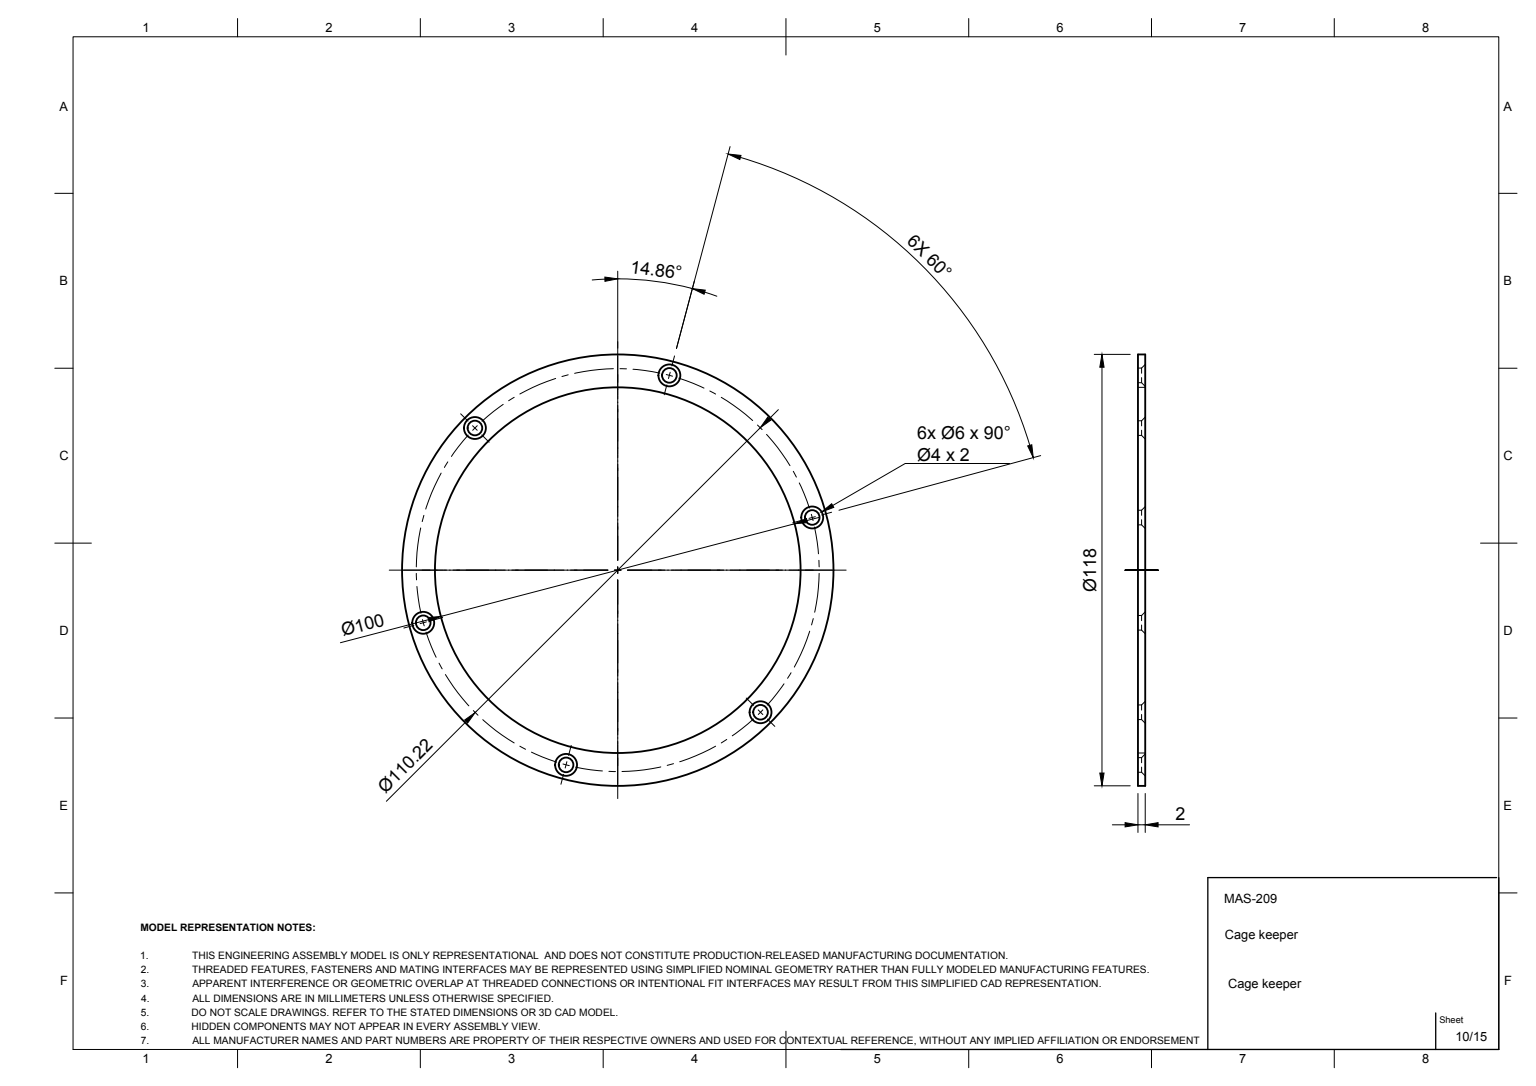
ISO-10303-21;
HEADER;
/* Generated by software containing ST-Developer
 * from STEP Tools, Inc. (www.steptools.com) 
 */

FILE_DESCRIPTION(
/* description */ ('Independent bearing-supported roller-ramp one-way clutch. Six logarit
hmic ramps with plain solid rollers, sprung guided plungers, native Co
il variants, removable shared keepers, rounded parallel key, shaft wit
h complete retaining lips, bronze journal/thrust support and bolted co
vers. Native rotor, roller planar/spin and plunger joints permit manua
l geometric engaged/released inspection. Automatic frictional torque s
witching/contact dynamics are not simulated; no capacity, hardness, fi
t, lubrication, speed, force or life rating. External input driver/cou
pling/anchors outside assembly.'),
/* implementation_level */ '2;1');

FILE_NAME(
/* name */ 'Cage keeper.step',
/* time_stamp */ '2026-11-08T07:04:38-08:00',
/* author */ (''),
/* organization */ (''),
/* preprocessor_version */ 'ST-DEVELOPER v20.2',
/* originating_system */ 'Autodesk Translation Framework v15.17.0.0',
/* authorisation */ '');

FILE_SCHEMA (('AUTOMOTIVE_DESIGN { 1 0 10303 214 3 1 1 }'));
ENDSEC;

DATA;
#10=MECHANICAL_DESIGN_GEOMETRIC_PRESENTATION_REPRESENTATION('',(#307),#99526);
#247=CONICAL_SURFACE('',#19556,2.5,0.785398163397448);
#248=CONICAL_SURFACE('',#19561,2.5,0.785398163397448);
#249=CONICAL_SURFACE('',#19566,2.5,0.785398163397448);
#250=CONICAL_SURFACE('',#19571,2.5,0.785398163397448);
#251=CONICAL_SURFACE('',#19576,2.5,0.785398163397448);
#252=CONICAL_SURFACE('',#19581,2.5,0.785398163397448);
#275=SHAPE_REPRESENTATION_RELATIONSHIP('SRR','None',#99632,#291);
#291=ADVANCED_BREP_SHAPE_REPRESENTATION('',(#323),#99517);
#307=STYLED_ITEM('',(#99715),#323);
#323=MANIFOLD_SOLID_BREP('Body1',#18277);
#416=FACE_BOUND('',#2646,.T.);
#417=FACE_BOUND('',#2647,.T.);
#418=FACE_BOUND('',#2648,.T.);
#419=FACE_BOUND('',#2649,.T.);
#420=FACE_BOUND('',#2650,.T.);
#421=FACE_BOUND('',#2651,.T.);
#422=FACE_BOUND('',#2652,.T.);
#423=FACE_BOUND('',#2654,.T.);
#424=FACE_BOUND('',#2655,.T.);
#425=FACE_BOUND('',#2656,.T.);
#426=FACE_BOUND('',#2657,.T.);
#427=FACE_BOUND('',#2658,.T.);
#428=FACE_BOUND('',#2659,.T.);
#429=FACE_BOUND('',#2660,.T.);
#577=PLANE('',#19592);
#578=PLANE('',#19593);
#1550=FACE_OUTER_BOUND('',#2631,.T.);
#1551=FACE_OUTER_BOUND('',#2632,.T.);
#1552=FACE_OUTER_BOUND('',#2633,.T.);
#1553=FACE_OUTER_BOUND('',#2634,.T.);
#1554=FACE_OUTER_BOUND('',#2635,.T.);
#1555=FACE_OUTER_BOUND('',#2636,.T.);
#1556=FACE_OUTER_BOUND('',#2637,.T.);
#1557=FACE_OUTER_BOUND('',#2638,.T.);
#1558=FACE_OUTER_BOUND('',#2639,.T.);
#1559=FACE_OUTER_BOUND('',#2640,.T.);
#1560=FACE_OUTER_BOUND('',#2641,.T.);
#1561=FACE_OUTER_BOUND('',#2642,.T.);
#1562=FACE_OUTER_BOUND('',#2643,.T.);
#1563=FACE_OUTER_BOUND('',#2644,.T.);
#1564=FACE_OUTER_BOUND('',#2645,.T.);
#1565=FACE_OUTER_BOUND('',#2653,.T.);
#2631=EDGE_LOOP('',(#15948,#15949,#15950,#15951));
#2632=EDGE_LOOP('',(#15952,#15953,#15954,#15955));
#2633=EDGE_LOOP('',(#15956,#15957,#15958,#15959));
#2634=EDGE_LOOP('',(#15960,#15961,#15962,#15963));
#2635=EDGE_LOOP('',(#15964,#15965,#15966,#15967));
#2636=EDGE_LOOP('',(#15968,#15969,#15970,#15971));
#2637=EDGE_LOOP('',(#15972,#15973,#15974,#15975));
#2638=EDGE_LOOP('',(#15976,#15977,#15978,#15979));
#2639=EDGE_LOOP('',(#15980,#15981,#15982,#15983));
#2640=EDGE_LOOP('',(#15984,#15985,#15986,#15987));
#2641=EDGE_LOOP('',(#15988,#15989,#15990,#15991));
#2642=EDGE_LOOP('',(#15992,#15993,#15994,#15995));
#2643=EDGE_LOOP('',(#15996,#15997,#15998,#15999));
#2644=EDGE_LOOP('',(#16000,#16001,#16002,#16003));
#2645=EDGE_LOOP('',(#16004));
#2646=EDGE_LOOP('',(#16005));
#2647=EDGE_LOOP('',(#16006));
#2648=EDGE_LOOP('',(#16007));
#2649=EDGE_LOOP('',(#16008));
#2650=EDGE_LOOP('',(#16009));
#2651=EDGE_LOOP('',(#16010));
#2652=EDGE_LOOP('',(#16011));
#2653=EDGE_LOOP('',(#16012));
#2654=EDGE_LOOP('',(#16013));
#2655=EDGE_LOOP('',(#16014));
#2656=EDGE_LOOP('',(#16015));
#2657=EDGE_LOOP('',(#16016));
#2658=EDGE_LOOP('',(#16017));
#2659=EDGE_LOOP('',(#16018));
#2660=EDGE_LOOP('',(#16019));
#3054=CIRCLE('',#19557,3.);
#3055=CIRCLE('',#19558,2.);
#3056=CIRCLE('',#19560,2.);
#3057=CIRCLE('',#19562,3.);
#3058=CIRCLE('',#19563,2.);
#3059=CIRCLE('',#19565,2.);
#3060=CIRCLE('',#19567,3.);
#3061=CIRCLE('',#19568,2.);
#3062=CIRCLE('',#19570,2.);
#3063=CIRCLE('',#19572,3.);
#3064=CIRCLE('',#19573,2.);
#3065=CIRCLE('',#19575,2.);
#3066=CIRCLE('',#19577,3.);
#3067=CIRCLE('',#19578,2.);
#3068=CIRCLE('',#19580,2.);
#3069=CIRCLE('',#19582,3.);
#3070=CIRCLE('',#19583,2.);
#3071=CIRCLE('',#19585,2.);
#3072=CIRCLE('',#19587,50.);
#3073=CIRCLE('',#19588,50.);
#3074=CIRCLE('',#19590,59.);
#3075=CIRCLE('',#19591,59.);
#5416=LINE('',#94779,#6320);
#5417=LINE('',#94783,#6321);
#5418=LINE('',#94789,#6322);
#5419=LINE('',#94793,#6323);
#5420=LINE('',#94799,#6324);
#5421=LINE('',#94803,#6325);
#5422=LINE('',#94809,#6326);
#5423=LINE('',#94813,#6327);
#5424=LINE('',#94819,#6328);
#5425=LINE('',#94823,#6329);
#5426=LINE('',#94829,#6330);
#5427=LINE('',#94833,#6331);
#5428=LINE('',#94839,#6332);
#5429=LINE('',#94845,#6333);
#6320=VECTOR('',#22775,2.5);
#6321=VECTOR('',#22780,2.);
#6322=VECTOR('',#22787,2.5);
#6323=VECTOR('',#22792,2.);
#6324=VECTOR('',#22799,2.5);
#6325=VECTOR('',#22804,2.);
#6326=VECTOR('',#22811,2.5);
#6327=VECTOR('',#22816,2.);
#6328=VECTOR('',#22823,2.5);
#6329=VECTOR('',#22828,2.);
#6330=VECTOR('',#22835,2.5);
#6331=VECTOR('',#22840,2.);
#6332=VECTOR('',#22847,50.);
#6333=VECTOR('',#22854,59.);
#8069=VERTEX_POINT('',#94776);
#8070=VERTEX_POINT('',#94778);
#8071=VERTEX_POINT('',#94782);
#8072=VERTEX_POINT('',#94786);
#8073=VERTEX_POINT('',#94788);
#8074=VERTEX_POINT('',#94792);
#8075=VERTEX_POINT('',#94796);
#8076=VERTEX_POINT('',#94798);
#8077=VERTEX_POINT('',#94802);
#8078=VERTEX_POINT('',#94806);
#8079=VERTEX_POINT('',#94808);
#8080=VERTEX_POINT('',#94812);
#8081=VERTEX_POINT('',#94816);
#8082=VERTEX_POINT('',#94818);
#8083=VERTEX_POINT('',#94822);
#8084=VERTEX_POINT('',#94826);
#8085=VERTEX_POINT('',#94828);
#8086=VERTEX_POINT('',#94832);
#8087=VERTEX_POINT('',#94836);
#8088=VERTEX_POINT('',#94838);
#8089=VERTEX_POINT('',#94842);
#8090=VERTEX_POINT('',#94844);
#10726=EDGE_CURVE('',#8069,#8069,#3054,.T.);
#10727=EDGE_CURVE('',#8069,#8070,#5416,.T.);
#10728=EDGE_CURVE('',#8070,#8070,#3055,.T.);
#10729=EDGE_CURVE('',#8070,#8071,#5417,.T.);
#10730=EDGE_CURVE('',#8071,#8071,#3056,.T.);
#10731=EDGE_CURVE('',#8072,#8072,#3057,.T.);
#10732=EDGE_CURVE('',#8072,#8073,#5418,.T.);
#10733=EDGE_CURVE('',#8073,#8073,#3058,.T.);
#10734=EDGE_CURVE('',#8073,#8074,#5419,.T.);
#10735=EDGE_CURVE('',#8074,#8074,#3059,.T.);
#10736=EDGE_CURVE('',#8075,#8075,#3060,.T.);
#10737=EDGE_CURVE('',#8075,#8076,#5420,.T.);
#10738=EDGE_CURVE('',#8076,#8076,#3061,.T.);
#10739=EDGE_CURVE('',#8076,#8077,#5421,.T.);
#10740=EDGE_CURVE('',#8077,#8077,#3062,.T.);
#10741=EDGE_CURVE('',#8078,#8078,#3063,.T.);
#10742=EDGE_CURVE('',#8078,#8079,#5422,.T.);
#10743=EDGE_CURVE('',#8079,#8079,#3064,.T.);
#10744=EDGE_CURVE('',#8079,#8080,#5423,.T.);
#10745=EDGE_CURVE('',#8080,#8080,#3065,.T.);
#10746=EDGE_CURVE('',#8081,#8081,#3066,.T.);
#10747=EDGE_CURVE('',#8081,#8082,#5424,.T.);
#10748=EDGE_CURVE('',#8082,#8082,#3067,.T.);
#10749=EDGE_CURVE('',#8082,#8083,#5425,.T.);
#10750=EDGE_CURVE('',#8083,#8083,#3068,.T.);
#10751=EDGE_CURVE('',#8084,#8084,#3069,.T.);
#10752=EDGE_CURVE('',#8084,#8085,#5426,.T.);
#10753=EDGE_CURVE('',#8085,#8085,#3070,.T.);
#10754=EDGE_CURVE('',#8085,#8086,#5427,.T.);
#10755=EDGE_CURVE('',#8086,#8086,#3071,.T.);
#10756=EDGE_CURVE('',#8087,#8087,#3072,.T.);
#10757=EDGE_CURVE('',#8087,#8088,#5428,.T.);
#10758=EDGE_CURVE('',#8088,#8088,#3073,.T.);
#10759=EDGE_CURVE('',#8089,#8089,#3074,.T.);
#10760=EDGE_CURVE('',#8089,#8090,#5429,.T.);
#10761=EDGE_CURVE('',#8090,#8090,#3075,.T.);
#15948=ORIENTED_EDGE('',*,*,#10726,.F.);
#15949=ORIENTED_EDGE('',*,*,#10727,.T.);
#15950=ORIENTED_EDGE('',*,*,#10728,.T.);
#15951=ORIENTED_EDGE('',*,*,#10727,.F.);
#15952=ORIENTED_EDGE('',*,*,#10728,.F.);
#15953=ORIENTED_EDGE('',*,*,#10729,.T.);
#15954=ORIENTED_EDGE('',*,*,#10730,.F.);
#15955=ORIENTED_EDGE('',*,*,#10729,.F.);
#15956=ORIENTED_EDGE('',*,*,#10731,.F.);
#15957=ORIENTED_EDGE('',*,*,#10732,.T.);
#15958=ORIENTED_EDGE('',*,*,#10733,.T.);
#15959=ORIENTED_EDGE('',*,*,#10732,.F.);
#15960=ORIENTED_EDGE('',*,*,#10733,.F.);
#15961=ORIENTED_EDGE('',*,*,#10734,.T.);
#15962=ORIENTED_EDGE('',*,*,#10735,.F.);
#15963=ORIENTED_EDGE('',*,*,#10734,.F.);
#15964=ORIENTED_EDGE('',*,*,#10736,.F.);
#15965=ORIENTED_EDGE('',*,*,#10737,.T.);
#15966=ORIENTED_EDGE('',*,*,#10738,.T.);
#15967=ORIENTED_EDGE('',*,*,#10737,.F.);
#15968=ORIENTED_EDGE('',*,*,#10738,.F.);
#15969=ORIENTED_EDGE('',*,*,#10739,.T.);
#15970=ORIENTED_EDGE('',*,*,#10740,.F.);
#15971=ORIENTED_EDGE('',*,*,#10739,.F.);
#15972=ORIENTED_EDGE('',*,*,#10741,.F.);
#15973=ORIENTED_EDGE('',*,*,#10742,.T.);
#15974=ORIENTED_EDGE('',*,*,#10743,.T.);
#15975=ORIENTED_EDGE('',*,*,#10742,.F.);
#15976=ORIENTED_EDGE('',*,*,#10743,.F.);
#15977=ORIENTED_EDGE('',*,*,#10744,.T.);
#15978=ORIENTED_EDGE('',*,*,#10745,.F.);
#15979=ORIENTED_EDGE('',*,*,#10744,.F.);
#15980=ORIENTED_EDGE('',*,*,#10746,.F.);
#15981=ORIENTED_EDGE('',*,*,#10747,.T.);
#15982=ORIENTED_EDGE('',*,*,#10748,.T.);
#15983=ORIENTED_EDGE('',*,*,#10747,.F.);
#15984=ORIENTED_EDGE('',*,*,#10748,.F.);
#15985=ORIENTED_EDGE('',*,*,#10749,.T.);
#15986=ORIENTED_EDGE('',*,*,#10750,.F.);
#15987=ORIENTED_EDGE('',*,*,#10749,.F.);
#15988=ORIENTED_EDGE('',*,*,#10751,.F.);
#15989=ORIENTED_EDGE('',*,*,#10752,.T.);
#15990=ORIENTED_EDGE('',*,*,#10753,.T.);
#15991=ORIENTED_EDGE('',*,*,#10752,.F.);
#15992=ORIENTED_EDGE('',*,*,#10753,.F.);
#15993=ORIENTED_EDGE('',*,*,#10754,.T.);
#15994=ORIENTED_EDGE('',*,*,#10755,.F.);
#15995=ORIENTED_EDGE('',*,*,#10754,.F.);
#15996=ORIENTED_EDGE('',*,*,#10756,.F.);
#15997=ORIENTED_EDGE('',*,*,#10757,.T.);
#15998=ORIENTED_EDGE('',*,*,#10758,.T.);
#15999=ORIENTED_EDGE('',*,*,#10757,.F.);
#16000=ORIENTED_EDGE('',*,*,#10759,.F.);
#16001=ORIENTED_EDGE('',*,*,#10760,.T.);
#16002=ORIENTED_EDGE('',*,*,#10761,.T.);
#16003=ORIENTED_EDGE('',*,*,#10760,.F.);
#16004=ORIENTED_EDGE('',*,*,#10759,.T.);
#16005=ORIENTED_EDGE('',*,*,#10756,.T.);
#16006=ORIENTED_EDGE('',*,*,#10751,.T.);
#16007=ORIENTED_EDGE('',*,*,#10746,.T.);
#16008=ORIENTED_EDGE('',*,*,#10741,.T.);
#16009=ORIENTED_EDGE('',*,*,#10736,.T.);
#16010=ORIENTED_EDGE('',*,*,#10731,.T.);
#16011=ORIENTED_EDGE('',*,*,#10726,.T.);
#16012=ORIENTED_EDGE('',*,*,#10761,.F.);
#16013=ORIENTED_EDGE('',*,*,#10758,.F.);
#16014=ORIENTED_EDGE('',*,*,#10755,.T.);
#16015=ORIENTED_EDGE('',*,*,#10750,.T.);
#16016=ORIENTED_EDGE('',*,*,#10745,.T.);
#16017=ORIENTED_EDGE('',*,*,#10740,.T.);
#16018=ORIENTED_EDGE('',*,*,#10735,.T.);
#16019=ORIENTED_EDGE('',*,*,#10730,.T.);
#17202=CYLINDRICAL_SURFACE('',#19559,2.);
#17203=CYLINDRICAL_SURFACE('',#19564,2.);
#17204=CYLINDRICAL_SURFACE('',#19569,2.);
#17205=CYLINDRICAL_SURFACE('',#19574,2.);
#17206=CYLINDRICAL_SURFACE('',#19579,2.);
#17207=CYLINDRICAL_SURFACE('',#19584,2.);
#17208=CYLINDRICAL_SURFACE('',#19586,50.);
#17209=CYLINDRICAL_SURFACE('',#19589,59.);
#18148=ADVANCED_FACE('',(#1550),#247,.F.);
#18149=ADVANCED_FACE('',(#1551),#17202,.F.);
#18150=ADVANCED_FACE('',(#1552),#248,.F.);
#18151=ADVANCED_FACE('',(#1553),#17203,.F.);
#18152=ADVANCED_FACE('',(#1554),#249,.F.);
#18153=ADVANCED_FACE('',(#1555),#17204,.F.);
#18154=ADVANCED_FACE('',(#1556),#250,.F.);
#18155=ADVANCED_FACE('',(#1557),#17205,.F.);
#18156=ADVANCED_FACE('',(#1558),#251,.F.);
#18157=ADVANCED_FACE('',(#1559),#17206,.F.);
#18158=ADVANCED_FACE('',(#1560),#252,.F.);
#18159=ADVANCED_FACE('',(#1561),#17207,.F.);
#18160=ADVANCED_FACE('',(#1562),#17208,.F.);
#18161=ADVANCED_FACE('',(#1563),#17209,.T.);
#18162=ADVANCED_FACE('',(#1564,#416,#417,#418,#419,#420,#421,#422),#577,
 .T.);
#18163=ADVANCED_FACE('',(#1565,#423,#424,#425,#426,#427,#428,#429),#578,
 .F.);
#18277=CLOSED_SHELL('',(#18148,#18149,#18150,#18151,#18152,#18153,#18154,
#18155,#18156,#18157,#18158,#18159,#18160,#18161,#18162,#18163));
#19555=AXIS2_PLACEMENT_3D('',#94774,#22769,#22770);
#19556=AXIS2_PLACEMENT_3D('',#94775,#22771,#22772);
#19557=AXIS2_PLACEMENT_3D('',#94777,#22773,#22774);
#19558=AXIS2_PLACEMENT_3D('',#94780,#22776,#22777);
#19559=AXIS2_PLACEMENT_3D('',#94781,#22778,#22779);
#19560=AXIS2_PLACEMENT_3D('',#94784,#22781,#22782);
#19561=AXIS2_PLACEMENT_3D('',#94785,#22783,#22784);
#19562=AXIS2_PLACEMENT_3D('',#94787,#22785,#22786);
#19563=AXIS2_PLACEMENT_3D('',#94790,#22788,#22789);
#19564=AXIS2_PLACEMENT_3D('',#94791,#22790,#22791);
#19565=AXIS2_PLACEMENT_3D('',#94794,#22793,#22794);
#19566=AXIS2_PLACEMENT_3D('',#94795,#22795,#22796);
#19567=AXIS2_PLACEMENT_3D('',#94797,#22797,#22798);
#19568=AXIS2_PLACEMENT_3D('',#94800,#22800,#22801);
#19569=AXIS2_PLACEMENT_3D('',#94801,#22802,#22803);
#19570=AXIS2_PLACEMENT_3D('',#94804,#22805,#22806);
#19571=AXIS2_PLACEMENT_3D('',#94805,#22807,#22808);
#19572=AXIS2_PLACEMENT_3D('',#94807,#22809,#22810);
#19573=AXIS2_PLACEMENT_3D('',#94810,#22812,#22813);
#19574=AXIS2_PLACEMENT_3D('',#94811,#22814,#22815);
#19575=AXIS2_PLACEMENT_3D('',#94814,#22817,#22818);
#19576=AXIS2_PLACEMENT_3D('',#94815,#22819,#22820);
#19577=AXIS2_PLACEMENT_3D('',#94817,#22821,#22822);
#19578=AXIS2_PLACEMENT_3D('',#94820,#22824,#22825);
#19579=AXIS2_PLACEMENT_3D('',#94821,#22826,#22827);
#19580=AXIS2_PLACEMENT_3D('',#94824,#22829,#22830);
#19581=AXIS2_PLACEMENT_3D('',#94825,#22831,#22832);
#19582=AXIS2_PLACEMENT_3D('',#94827,#22833,#22834);
#19583=AXIS2_PLACEMENT_3D('',#94830,#22836,#22837);
#19584=AXIS2_PLACEMENT_3D('',#94831,#22838,#22839);
#19585=AXIS2_PLACEMENT_3D('',#94834,#22841,#22842);
#19586=AXIS2_PLACEMENT_3D('',#94835,#22843,#22844);
#19587=AXIS2_PLACEMENT_3D('',#94837,#22845,#22846);
#19588=AXIS2_PLACEMENT_3D('',#94840,#22848,#22849);
#19589=AXIS2_PLACEMENT_3D('',#94841,#22850,#22851);
#19590=AXIS2_PLACEMENT_3D('',#94843,#22852,#22853);
#19591=AXIS2_PLACEMENT_3D('',#94846,#22855,#22856);
#19592=AXIS2_PLACEMENT_3D('',#94847,#22857,#22858);
#19593=AXIS2_PLACEMENT_3D('',#94848,#22859,#22860);
#22769=DIRECTION('axis',(0.,0.,1.));
#22770=DIRECTION('refdir',(1.,0.,0.));
#22771=DIRECTION('center_axis',(0.,0.,1.));
#22772=DIRECTION('ref_axis',(1.,0.,0.));
#22773=DIRECTION('center_axis',(0.,0.,-1.));
#22774=DIRECTION('ref_axis',(1.,0.,0.));
#22775=DIRECTION('',(0.707106781186547,-8.65956056235493E-17,-0.707106781186548));
#22776=DIRECTION('center_axis',(0.,0.,-1.));
#22777=DIRECTION('ref_axis',(1.,0.,0.));
#22778=DIRECTION('center_axis',(0.,0.,-1.));
#22779=DIRECTION('ref_axis',(1.,0.,0.));
#22780=DIRECTION('',(0.,0.,-1.));
#22781=DIRECTION('center_axis',(0.,0.,1.));
#22782=DIRECTION('ref_axis',(1.,0.,0.));
#22783=DIRECTION('center_axis',(0.,0.,1.));
#22784=DIRECTION('ref_axis',(1.,0.,0.));
#22785=DIRECTION('center_axis',(0.,0.,-1.));
#22786=DIRECTION('ref_axis',(1.,0.,0.));
#22787=DIRECTION('',(0.707106781186547,-8.65956056235493E-17,-0.707106781186548));
#22788=DIRECTION('center_axis',(0.,0.,-1.));
#22789=DIRECTION('ref_axis',(1.,0.,0.));
#22790=DIRECTION('center_axis',(0.,0.,-1.));
#22791=DIRECTION('ref_axis',(1.,0.,0.));
#22792=DIRECTION('',(0.,0.,-1.));
#22793=DIRECTION('center_axis',(0.,0.,1.));
#22794=DIRECTION('ref_axis',(1.,0.,0.));
#22795=DIRECTION('center_axis',(0.,0.,1.));
#22796=DIRECTION('ref_axis',(1.,0.,0.));
#22797=DIRECTION('center_axis',(0.,0.,-1.));
#22798=DIRECTION('ref_axis',(1.,0.,0.));
#22799=DIRECTION('',(0.707106781186547,-8.65956056235493E-17,-0.707106781186548));
#22800=DIRECTION('center_axis',(0.,0.,-1.));
#22801=DIRECTION('ref_axis',(1.,0.,0.));
#22802=DIRECTION('center_axis',(0.,0.,-1.));
#22803=DIRECTION('ref_axis',(1.,0.,0.));
#22804=DIRECTION('',(0.,0.,-1.));
#22805=DIRECTION('center_axis',(0.,0.,1.));
#22806=DIRECTION('ref_axis',(1.,0.,0.));
#22807=DIRECTION('center_axis',(0.,0.,1.));
#22808=DIRECTION('ref_axis',(1.,0.,0.));
#22809=DIRECTION('center_axis',(0.,0.,-1.));
#22810=DIRECTION('ref_axis',(1.,0.,0.));
#22811=DIRECTION('',(0.707106781186547,-8.65956056235493E-17,-0.707106781186548));
#22812=DIRECTION('center_axis',(0.,0.,-1.));
#22813=DIRECTION('ref_axis',(1.,0.,0.));
#22814=DIRECTION('center_axis',(0.,0.,-1.));
#22815=DIRECTION('ref_axis',(1.,0.,0.));
#22816=DIRECTION('',(0.,0.,-1.));
#22817=DIRECTION('center_axis',(0.,0.,1.));
#22818=DIRECTION('ref_axis',(1.,0.,0.));
#22819=DIRECTION('center_axis',(0.,0.,1.));
#22820=DIRECTION('ref_axis',(1.,0.,0.));
#22821=DIRECTION('center_axis',(0.,0.,-1.));
#22822=DIRECTION('ref_axis',(1.,0.,0.));
#22823=DIRECTION('',(0.707106781186547,-8.65956056235493E-17,-0.707106781186548));
#22824=DIRECTION('center_axis',(0.,0.,-1.));
#22825=DIRECTION('ref_axis',(1.,0.,0.));
#22826=DIRECTION('center_axis',(0.,0.,-1.));
#22827=DIRECTION('ref_axis',(1.,0.,0.));
#22828=DIRECTION('',(0.,0.,-1.));
#22829=DIRECTION('center_axis',(0.,0.,1.));
#22830=DIRECTION('ref_axis',(1.,0.,0.));
#22831=DIRECTION('center_axis',(0.,0.,1.));
#22832=DIRECTION('ref_axis',(1.,0.,0.));
#22833=DIRECTION('center_axis',(0.,0.,-1.));
#22834=DIRECTION('ref_axis',(1.,0.,0.));
#22835=DIRECTION('',(0.707106781186547,-8.65956056235493E-17,-0.707106781186548));
#22836=DIRECTION('center_axis',(0.,0.,-1.));
#22837=DIRECTION('ref_axis',(1.,0.,0.));
#22838=DIRECTION('center_axis',(0.,0.,-1.));
#22839=DIRECTION('ref_axis',(1.,0.,0.));
#22840=DIRECTION('',(0.,0.,-1.));
#22841=DIRECTION('center_axis',(0.,0.,1.));
#22842=DIRECTION('ref_axis',(1.,0.,0.));
#22843=DIRECTION('center_axis',(0.,0.,1.));
#22844=DIRECTION('ref_axis',(1.,0.,0.));
#22845=DIRECTION('center_axis',(0.,0.,-1.));
#22846=DIRECTION('ref_axis',(1.,0.,0.));
#22847=DIRECTION('',(0.,0.,-1.));
#22848=DIRECTION('center_axis',(0.,0.,-1.));
#22849=DIRECTION('ref_axis',(1.,0.,0.));
#22850=DIRECTION('center_axis',(0.,0.,1.));
#22851=DIRECTION('ref_axis',(1.,0.,0.));
#22852=DIRECTION('center_axis',(0.,0.,1.));
#22853=DIRECTION('ref_axis',(1.,0.,0.));
#22854=DIRECTION('',(0.,0.,-1.));
#22855=DIRECTION('center_axis',(0.,0.,1.));
#22856=DIRECTION('ref_axis',(1.,0.,0.));
#22857=DIRECTION('center_axis',(0.,0.,1.));
#22858=DIRECTION('ref_axis',(1.,0.,0.));
#22859=DIRECTION('center_axis',(0.,0.,1.));
#22860=DIRECTION('ref_axis',(1.,0.,0.));
#94774=CARTESIAN_POINT('',(0.,0.,0.));
#94775=CARTESIAN_POINT('Origin',(-14.1292828945603,-53.2669068454841,1.5));
#94776=CARTESIAN_POINT('',(-17.1292828945603,-53.2669068454841,2.));
#94777=CARTESIAN_POINT('Origin',(-14.1292828945603,-53.2669068454841,2.));
#94778=CARTESIAN_POINT('',(-16.1292828945603,-53.2669068454841,1.));
#94779=CARTESIAN_POINT('',(-16.6292828945603,-53.2669068454841,1.5));
#94780=CARTESIAN_POINT('Origin',(-14.1292828945603,-53.2669068454841,1.));
#94781=CARTESIAN_POINT('Origin',(-14.1292828945603,-53.2669068454841,1.));
#94782=CARTESIAN_POINT('',(-16.1292828945603,-53.2669068454841,0.));
#94783=CARTESIAN_POINT('',(-16.1292828945603,-53.2669068454841,1.));
#94784=CARTESIAN_POINT('Origin',(-14.1292828945603,-53.2669068454841,0.));
#94785=CARTESIAN_POINT('Origin',(-39.0658530619283,38.8697713466882,1.5));
#94786=CARTESIAN_POINT('',(-42.0658530619283,38.8697713466882,2.));
#94787=CARTESIAN_POINT('Origin',(-39.0658530619283,38.8697713466882,2.));
#94788=CARTESIAN_POINT('',(-41.0658530619283,38.8697713466882,1.));
#94789=CARTESIAN_POINT('',(-41.5658530619283,38.8697713466882,1.5));
#94790=CARTESIAN_POINT('Origin',(-39.0658530619283,38.8697713466882,1.));
#94791=CARTESIAN_POINT('Origin',(-39.0658530619283,38.8697713466882,1.));
#94792=CARTESIAN_POINT('',(-41.0658530619283,38.8697713466882,0.));
#94793=CARTESIAN_POINT('',(-41.0658530619283,38.8697713466882,1.));
#94794=CARTESIAN_POINT('Origin',(-39.0658530619283,38.8697713466882,0.));
#94795=CARTESIAN_POINT('Origin',(53.1951359564886,14.3971354987959,1.5));
#94796=CARTESIAN_POINT('',(50.1951359564886,14.3971354987959,2.));
#94797=CARTESIAN_POINT('Origin',(53.1951359564886,14.3971354987959,2.));
#94798=CARTESIAN_POINT('',(51.1951359564886,14.3971354987959,1.));
#94799=CARTESIAN_POINT('',(50.6951359564886,14.3971354987959,1.5));
#94800=CARTESIAN_POINT('Origin',(53.1951359564886,14.3971354987959,1.));
#94801=CARTESIAN_POINT('Origin',(53.1951359564886,14.3971354987959,1.));
#94802=CARTESIAN_POINT('',(51.1951359564886,14.3971354987959,0.));
#94803=CARTESIAN_POINT('',(51.1951359564886,14.3971354987959,1.));
#94804=CARTESIAN_POINT('Origin',(53.1951359564886,14.3971354987959,0.));
#94805=CARTESIAN_POINT('Origin',(14.1292828945603,53.2669068454841,1.5));
#94806=CARTESIAN_POINT('',(11.1292828945603,53.2669068454841,2.));
#94807=CARTESIAN_POINT('Origin',(14.1292828945603,53.2669068454841,2.));
#94808=CARTESIAN_POINT('',(12.1292828945603,53.2669068454841,1.));
#94809=CARTESIAN_POINT('',(11.6292828945603,53.2669068454841,1.5));
#94810=CARTESIAN_POINT('Origin',(14.1292828945603,53.2669068454841,1.));
#94811=CARTESIAN_POINT('Origin',(14.1292828945603,53.2669068454841,1.));
#94812=CARTESIAN_POINT('',(12.1292828945603,53.2669068454841,0.));
#94813=CARTESIAN_POINT('',(12.1292828945603,53.2669068454841,1.));
#94814=CARTESIAN_POINT('Origin',(14.1292828945603,53.2669068454841,0.));
#94815=CARTESIAN_POINT('Origin',(-53.1951359564886,-14.3971354987959,1.5));
#94816=CARTESIAN_POINT('',(-56.1951359564886,-14.3971354987959,2.));
#94817=CARTESIAN_POINT('Origin',(-53.1951359564886,-14.3971354987959,2.));
#94818=CARTESIAN_POINT('',(-55.1951359564886,-14.3971354987959,1.));
#94819=CARTESIAN_POINT('',(-55.6951359564886,-14.3971354987959,1.5));
#94820=CARTESIAN_POINT('Origin',(-53.1951359564886,-14.3971354987959,1.));
#94821=CARTESIAN_POINT('Origin',(-53.1951359564886,-14.3971354987959,1.));
#94822=CARTESIAN_POINT('',(-55.1951359564886,-14.3971354987959,0.));
#94823=CARTESIAN_POINT('',(-55.1951359564886,-14.3971354987959,1.));
#94824=CARTESIAN_POINT('Origin',(-53.1951359564886,-14.3971354987959,0.));
#94825=CARTESIAN_POINT('Origin',(39.0658530619283,-38.8697713466882,1.5));
#94826=CARTESIAN_POINT('',(36.0658530619283,-38.8697713466882,2.));
#94827=CARTESIAN_POINT('Origin',(39.0658530619283,-38.8697713466882,2.));
#94828=CARTESIAN_POINT('',(37.0658530619283,-38.8697713466882,0.999999999999996));
#94829=CARTESIAN_POINT('',(36.5658530619283,-38.8697713466882,1.5));
#94830=CARTESIAN_POINT('Origin',(39.0658530619283,-38.8697713466882,1.));
#94831=CARTESIAN_POINT('Origin',(39.0658530619283,-38.8697713466882,1.));
#94832=CARTESIAN_POINT('',(37.0658530619283,-38.8697713466882,0.));
#94833=CARTESIAN_POINT('',(37.0658530619283,-38.8697713466882,1.));
#94834=CARTESIAN_POINT('Origin',(39.0658530619283,-38.8697713466882,0.));
#94835=CARTESIAN_POINT('Origin',(0.,0.,0.));
#94836=CARTESIAN_POINT('',(-50.,-6.12323399573677E-15,2.));
#94837=CARTESIAN_POINT('Origin',(0.,0.,2.));
#94838=CARTESIAN_POINT('',(-50.,-6.12323399573677E-15,0.));
#94839=CARTESIAN_POINT('',(-50.,-6.12323399573677E-15,0.));
#94840=CARTESIAN_POINT('Origin',(0.,0.,0.));
#94841=CARTESIAN_POINT('Origin',(0.,0.,0.));
#94842=CARTESIAN_POINT('',(-59.,-7.22541611496938E-15,2.));
#94843=CARTESIAN_POINT('Origin',(0.,0.,2.));
#94844=CARTESIAN_POINT('',(-59.,-7.22541611496938E-15,0.));
#94845=CARTESIAN_POINT('',(-59.,-7.22541611496938E-15,0.));
#94846=CARTESIAN_POINT('Origin',(0.,0.,0.));
#94847=CARTESIAN_POINT('Origin',(0.,0.,2.));
#94848=CARTESIAN_POINT('Origin',(0.,0.,0.));
#99499=UNCERTAINTY_MEASURE_WITH_UNIT(LENGTH_MEASURE(0.01),#99527,
'DISTANCE_ACCURACY_VALUE',
'Maximum model space distance between geometric entities at asserted c
onnectivities');
#99508=UNCERTAINTY_MEASURE_WITH_UNIT(LENGTH_MEASURE(0.01),#99527,
'DISTANCE_ACCURACY_VALUE',
'Maximum model space distance between geometric entities at asserted c
onnectivities');
#99517=(
GEOMETRIC_REPRESENTATION_CONTEXT(3)
GLOBAL_UNCERTAINTY_ASSIGNED_CONTEXT((#99499))
GLOBAL_UNIT_ASSIGNED_CONTEXT((#99527,#99529,#99530))
REPRESENTATION_CONTEXT('','3D')
);
#99526=(
GEOMETRIC_REPRESENTATION_CONTEXT(3)
GLOBAL_UNCERTAINTY_ASSIGNED_CONTEXT((#99508))
GLOBAL_UNIT_ASSIGNED_CONTEXT((#99527,#99529,#99530))
REPRESENTATION_CONTEXT('','3D')
);
#99527=(
LENGTH_UNIT()
NAMED_UNIT(*)
SI_UNIT(.MILLI.,.METRE.)
);
#99529=(
NAMED_UNIT(*)
PLANE_ANGLE_UNIT()
SI_UNIT($,.RADIAN.)
);
#99530=(
NAMED_UNIT(*)
SI_UNIT($,.STERADIAN.)
SOLID_ANGLE_UNIT()
);
#99539=SHAPE_DEFINITION_REPRESENTATION(#99556,#99632);
#99556=PRODUCT_DEFINITION_SHAPE('',$,#99650);
#99632=SHAPE_REPRESENTATION('',(#19555),#99517);
#99641=PRODUCT_DEFINITION_CONTEXT('part definition',#99694,'design');
#99650=PRODUCT_DEFINITION('Cage keeper','Cage keeper',#99667,#99641);
#99667=PRODUCT_DEFINITION_FORMATION('',$,#99704);
#99694=APPLICATION_CONTEXT(
'Core Data for Automotive Mechanical Design Process');
#99695=PRODUCT_CONTEXT('part definition',#99694,'mechanical');
#99704=PRODUCT('Cage keeper','Cage keeper',$,(#99695));
#99715=PRESENTATION_STYLE_ASSIGNMENT((#99728));
#99728=SURFACE_STYLE_USAGE(.BOTH.,#99741);
#99741=SURFACE_SIDE_STYLE('',(#99754));
#99754=SURFACE_STYLE_FILL_AREA(#99767);
#99767=FILL_AREA_STYLE('Light blue',(#99780));
#99780=FILL_AREA_STYLE_COLOUR('Light blue',#99793);
#99793=COLOUR_RGB('Light blue',0.662745098039216,0.831372549019608,0.949019607843137);
ENDSEC;
END-ISO-10303-21;
